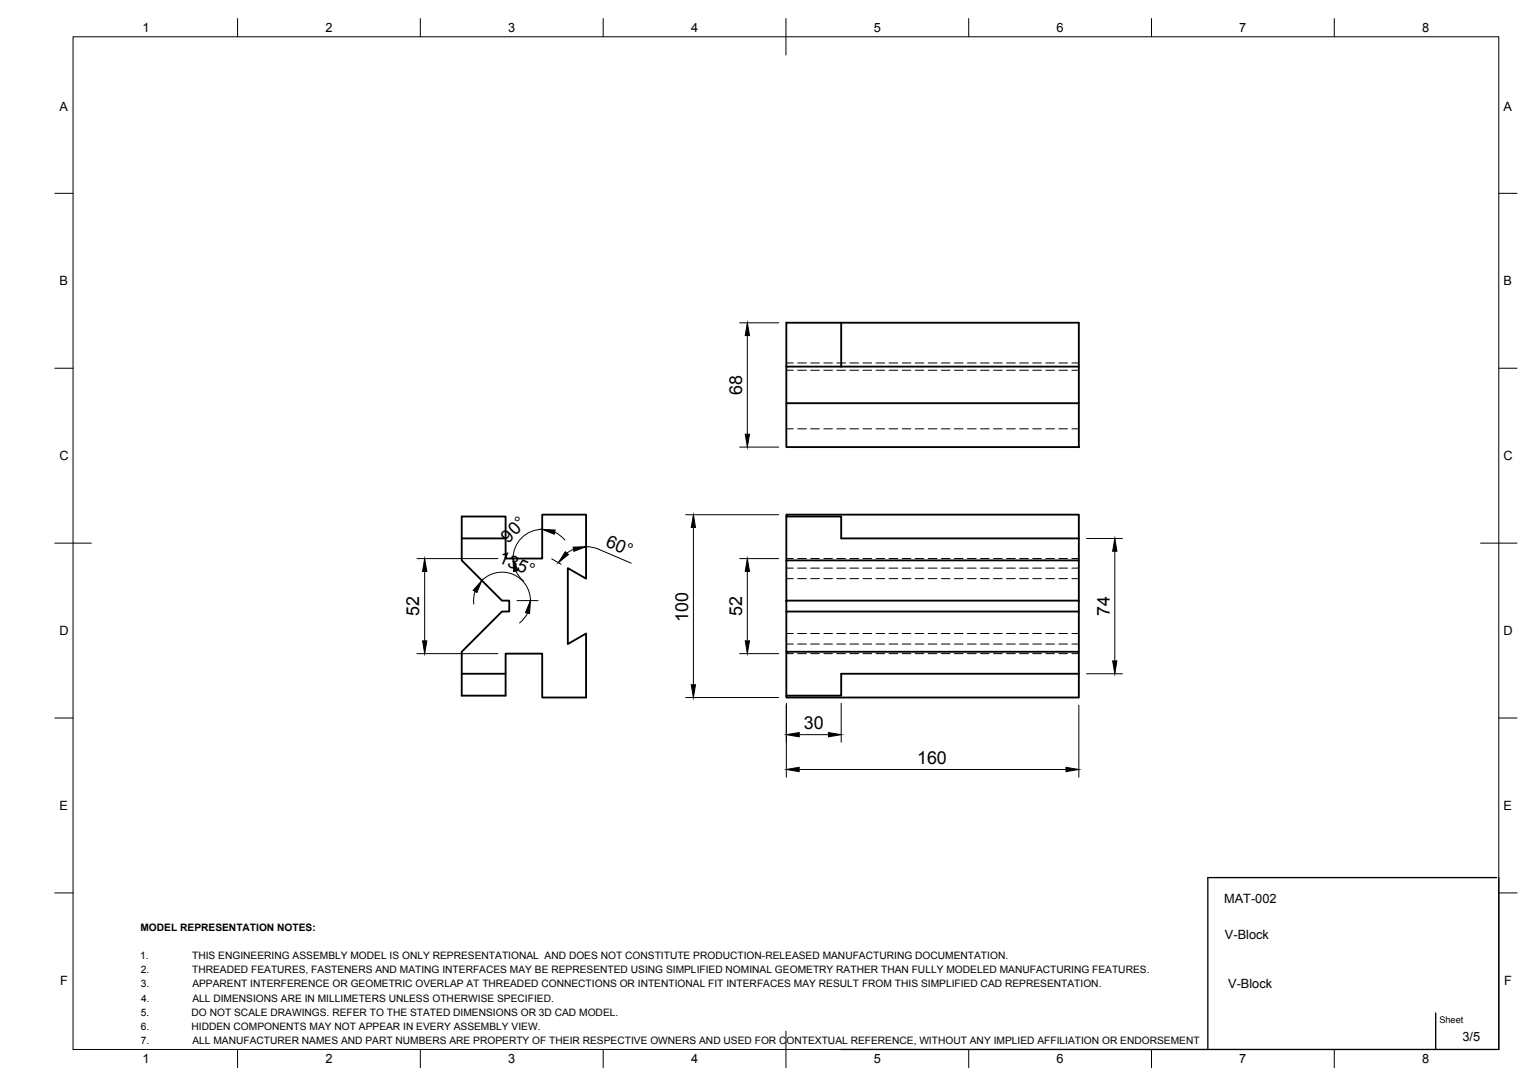
ISO-10303-21;
HEADER;
/* Generated by software containing ST-Developer
 * from STEP Tools, Inc. (www.steptools.com) 
 */

FILE_DESCRIPTION(
/* description */ ('STEP AP214'),
/* implementation_level */ '2;1');

FILE_NAME(
/* name */ 'V-Block.step',
/* time_stamp */ '2026-11-14T04:35:10-08:00',
/* author */ (''),
/* organization */ (''),
/* preprocessor_version */ 'ST-DEVELOPER v20.2',
/* originating_system */ 'Autodesk Translation Framework v15.17.0.0',
/* authorisation */ '');

FILE_SCHEMA (('AUTOMOTIVE_DESIGN { 1 0 10303 214 3 1 1 }'));
ENDSEC;

DATA;
#10=MECHANICAL_DESIGN_GEOMETRIC_PRESENTATION_REPRESENTATION('',(#107),#2477);
#99=SHAPE_REPRESENTATION_RELATIONSHIP('SRR','None',#2497,#103);
#103=ADVANCED_BREP_SHAPE_REPRESENTATION('',(#111),#2473);
#107=STYLED_ITEM('',(#2526),#111);
#111=MANIFOLD_SOLID_BREP('Body1',#1427);
#115=FACE_OUTER_BOUND('',#194,.T.);
#116=FACE_OUTER_BOUND('',#195,.T.);
#117=FACE_OUTER_BOUND('',#196,.T.);
#118=FACE_OUTER_BOUND('',#197,.T.);
#119=FACE_OUTER_BOUND('',#198,.T.);
#120=FACE_OUTER_BOUND('',#199,.T.);
#121=FACE_OUTER_BOUND('',#200,.T.);
#122=FACE_OUTER_BOUND('',#201,.T.);
#123=FACE_OUTER_BOUND('',#202,.T.);
#124=FACE_OUTER_BOUND('',#203,.T.);
#125=FACE_OUTER_BOUND('',#204,.T.);
#126=FACE_OUTER_BOUND('',#205,.T.);
#127=FACE_OUTER_BOUND('',#206,.T.);
#128=FACE_OUTER_BOUND('',#207,.T.);
#129=FACE_OUTER_BOUND('',#208,.T.);
#130=FACE_OUTER_BOUND('',#209,.T.);
#131=FACE_OUTER_BOUND('',#210,.T.);
#132=FACE_OUTER_BOUND('',#211,.T.);
#133=FACE_OUTER_BOUND('',#212,.T.);
#134=FACE_OUTER_BOUND('',#213,.T.);
#135=FACE_OUTER_BOUND('',#214,.T.);
#136=FACE_OUTER_BOUND('',#215,.T.);
#137=FACE_OUTER_BOUND('',#216,.T.);
#138=FACE_OUTER_BOUND('',#217,.T.);
#139=FACE_OUTER_BOUND('',#218,.T.);
#140=FACE_OUTER_BOUND('',#219,.T.);
#141=FACE_OUTER_BOUND('',#220,.T.);
#142=FACE_OUTER_BOUND('',#221,.T.);
#194=EDGE_LOOP('',(#894,#895,#896,#897));
#195=EDGE_LOOP('',(#898,#899,#900,#901));
#196=EDGE_LOOP('',(#902,#903,#904,#905));
#197=EDGE_LOOP('',(#906,#907,#908,#909));
#198=EDGE_LOOP('',(#910,#911,#912,#913));
#199=EDGE_LOOP('',(#914,#915,#916,#917,#918,#919));
#200=EDGE_LOOP('',(#920,#921,#922,#923,#924,#925));
#201=EDGE_LOOP('',(#926,#927,#928,#929));
#202=EDGE_LOOP('',(#930,#931,#932,#933));
#203=EDGE_LOOP('',(#934,#935,#936,#937));
#204=EDGE_LOOP('',(#938,#939,#940,#941));
#205=EDGE_LOOP('',(#942,#943,#944,#945));
#206=EDGE_LOOP('',(#946,#947,#948,#949,#950,#951));
#207=EDGE_LOOP('',(#952,#953,#954,#955,#956,#957));
#208=EDGE_LOOP('',(#958,#959,#960,#961));
#209=EDGE_LOOP('',(#962,#963,#964,#965));
#210=EDGE_LOOP('',(#966,#967,#968,#969));
#211=EDGE_LOOP('',(#970,#971,#972,#973));
#212=EDGE_LOOP('',(#974,#975,#976,#977));
#213=EDGE_LOOP('',(#978,#979,#980,#981));
#214=EDGE_LOOP('',(#982,#983,#984,#985));
#215=EDGE_LOOP('',(#986,#987,#988,#989));
#216=EDGE_LOOP('',(#990,#991,#992,#993,#994,#995,#996,#997,#998,#999,#1000,
#1001,#1002,#1003,#1004,#1005,#1006,#1007,#1008,#1009,#1010,#1011));
#217=EDGE_LOOP('',(#1012,#1013,#1014,#1015,#1016,#1017,#1018,#1019,#1020,
#1021,#1022,#1023,#1024,#1025,#1026,#1027,#1028,#1029,#1030,#1031,#1032,
#1033));
#218=EDGE_LOOP('',(#1034,#1035,#1036,#1037));
#219=EDGE_LOOP('',(#1038,#1039,#1040,#1041));
#220=EDGE_LOOP('',(#1042,#1043,#1044,#1045));
#221=EDGE_LOOP('',(#1046,#1047,#1048,#1049));
#276=LINE('',#2000,#423);
#277=LINE('',#2002,#424);
#278=LINE('',#2004,#425);
#279=LINE('',#2005,#426);
#280=LINE('',#2009,#427);
#281=LINE('',#2011,#428);
#282=LINE('',#2013,#429);
#283=LINE('',#2014,#430);
#284=LINE('',#2018,#431);
#285=LINE('',#2020,#432);
#286=LINE('',#2022,#433);
#287=LINE('',#2023,#434);
#288=LINE('',#2026,#435);
#289=LINE('',#2028,#436);
#290=LINE('',#2029,#437);
#291=LINE('',#2032,#438);
#292=LINE('',#2034,#439);
#293=LINE('',#2035,#440);
#294=LINE('',#2037,#441);
#295=LINE('',#2039,#442);
#296=LINE('',#2041,#443);
#297=LINE('',#2042,#444);
#298=LINE('',#2045,#445);
#299=LINE('',#2047,#446);
#300=LINE('',#2049,#447);
#301=LINE('',#2051,#448);
#302=LINE('',#2052,#449);
#303=LINE('',#2055,#450);
#304=LINE('',#2057,#451);
#305=LINE('',#2058,#452);
#306=LINE('',#2061,#453);
#307=LINE('',#2063,#454);
#308=LINE('',#2064,#455);
#309=LINE('',#2067,#456);
#310=LINE('',#2069,#457);
#311=LINE('',#2070,#458);
#312=LINE('',#2073,#459);
#313=LINE('',#2075,#460);
#314=LINE('',#2076,#461);
#315=LINE('',#2079,#462);
#316=LINE('',#2081,#463);
#317=LINE('',#2082,#464);
#318=LINE('',#2084,#465);
#319=LINE('',#2086,#466);
#320=LINE('',#2088,#467);
#321=LINE('',#2089,#468);
#322=LINE('',#2092,#469);
#323=LINE('',#2094,#470);
#324=LINE('',#2096,#471);
#325=LINE('',#2098,#472);
#326=LINE('',#2099,#473);
#327=LINE('',#2102,#474);
#328=LINE('',#2104,#475);
#329=LINE('',#2105,#476);
#330=LINE('',#2108,#477);
#331=LINE('',#2110,#478);
#332=LINE('',#2111,#479);
#333=LINE('',#2114,#480);
#334=LINE('',#2116,#481);
#335=LINE('',#2117,#482);
#336=LINE('',#2120,#483);
#337=LINE('',#2122,#484);
#338=LINE('',#2123,#485);
#339=LINE('',#2126,#486);
#340=LINE('',#2128,#487);
#341=LINE('',#2129,#488);
#342=LINE('',#2132,#489);
#343=LINE('',#2134,#490);
#344=LINE('',#2135,#491);
#345=LINE('',#2138,#492);
#346=LINE('',#2140,#493);
#347=LINE('',#2141,#494);
#348=LINE('',#2143,#495);
#349=LINE('',#2144,#496);
#350=LINE('',#2146,#497);
#351=LINE('',#2147,#498);
#352=LINE('',#2150,#499);
#353=LINE('',#2153,#500);
#423=VECTOR('',#1606,1000.);
#424=VECTOR('',#1607,1000.);
#425=VECTOR('',#1608,1000.);
#426=VECTOR('',#1609,1000.);
#427=VECTOR('',#1612,1000.);
#428=VECTOR('',#1613,1000.);
#429=VECTOR('',#1614,1000.);
#430=VECTOR('',#1615,1000.);
#431=VECTOR('',#1618,1000.);
#432=VECTOR('',#1619,1000.);
#433=VECTOR('',#1620,1000.);
#434=VECTOR('',#1621,1000.);
#435=VECTOR('',#1624,1000.);
#436=VECTOR('',#1625,1000.);
#437=VECTOR('',#1626,1000.);
#438=VECTOR('',#1629,1000.);
#439=VECTOR('',#1630,1000.);
#440=VECTOR('',#1631,1000.);
#441=VECTOR('',#1634,1000.);
#442=VECTOR('',#1635,1000.);
#443=VECTOR('',#1636,1000.);
#444=VECTOR('',#1637,1000.);
#445=VECTOR('',#1640,1000.);
#446=VECTOR('',#1641,1000.);
#447=VECTOR('',#1642,1000.);
#448=VECTOR('',#1643,1000.);
#449=VECTOR('',#1644,1000.);
#450=VECTOR('',#1647,1000.);
#451=VECTOR('',#1648,1000.);
#452=VECTOR('',#1649,1000.);
#453=VECTOR('',#1652,1000.);
#454=VECTOR('',#1653,1000.);
#455=VECTOR('',#1654,1000.);
#456=VECTOR('',#1657,1000.);
#457=VECTOR('',#1658,1000.);
#458=VECTOR('',#1659,1000.);
#459=VECTOR('',#1662,1000.);
#460=VECTOR('',#1663,1000.);
#461=VECTOR('',#1664,1000.);
#462=VECTOR('',#1667,1000.);
#463=VECTOR('',#1668,1000.);
#464=VECTOR('',#1669,1000.);
#465=VECTOR('',#1672,1000.);
#466=VECTOR('',#1673,1000.);
#467=VECTOR('',#1674,1000.);
#468=VECTOR('',#1675,1000.);
#469=VECTOR('',#1678,1000.);
#470=VECTOR('',#1679,1000.);
#471=VECTOR('',#1680,1000.);
#472=VECTOR('',#1681,1000.);
#473=VECTOR('',#1682,1000.);
#474=VECTOR('',#1685,1000.);
#475=VECTOR('',#1686,1000.);
#476=VECTOR('',#1687,1000.);
#477=VECTOR('',#1690,1000.);
#478=VECTOR('',#1691,1000.);
#479=VECTOR('',#1692,1000.);
#480=VECTOR('',#1695,1000.);
#481=VECTOR('',#1696,1000.);
#482=VECTOR('',#1697,1000.);
#483=VECTOR('',#1700,1000.);
#484=VECTOR('',#1701,1000.);
#485=VECTOR('',#1702,1000.);
#486=VECTOR('',#1705,1000.);
#487=VECTOR('',#1706,1000.);
#488=VECTOR('',#1707,1000.);
#489=VECTOR('',#1710,1000.);
#490=VECTOR('',#1711,1000.);
#491=VECTOR('',#1712,1000.);
#492=VECTOR('',#1715,1000.);
#493=VECTOR('',#1716,1000.);
#494=VECTOR('',#1717,1000.);
#495=VECTOR('',#1720,1000.);
#496=VECTOR('',#1721,1000.);
#497=VECTOR('',#1724,1000.);
#498=VECTOR('',#1725,1000.);
#499=VECTOR('',#1730,1000.);
#500=VECTOR('',#1735,1000.);
#570=VERTEX_POINT('',#1998);
#571=VERTEX_POINT('',#1999);
#572=VERTEX_POINT('',#2001);
#573=VERTEX_POINT('',#2003);
#574=VERTEX_POINT('',#2007);
#575=VERTEX_POINT('',#2008);
#576=VERTEX_POINT('',#2010);
#577=VERTEX_POINT('',#2012);
#578=VERTEX_POINT('',#2016);
#579=VERTEX_POINT('',#2017);
#580=VERTEX_POINT('',#2019);
#581=VERTEX_POINT('',#2021);
#582=VERTEX_POINT('',#2025);
#583=VERTEX_POINT('',#2027);
#584=VERTEX_POINT('',#2031);
#585=VERTEX_POINT('',#2033);
#586=VERTEX_POINT('',#2038);
#587=VERTEX_POINT('',#2040);
#588=VERTEX_POINT('',#2044);
#589=VERTEX_POINT('',#2046);
#590=VERTEX_POINT('',#2048);
#591=VERTEX_POINT('',#2050);
#592=VERTEX_POINT('',#2054);
#593=VERTEX_POINT('',#2056);
#594=VERTEX_POINT('',#2060);
#595=VERTEX_POINT('',#2062);
#596=VERTEX_POINT('',#2066);
#597=VERTEX_POINT('',#2068);
#598=VERTEX_POINT('',#2072);
#599=VERTEX_POINT('',#2074);
#600=VERTEX_POINT('',#2078);
#601=VERTEX_POINT('',#2080);
#602=VERTEX_POINT('',#2085);
#603=VERTEX_POINT('',#2087);
#604=VERTEX_POINT('',#2091);
#605=VERTEX_POINT('',#2093);
#606=VERTEX_POINT('',#2095);
#607=VERTEX_POINT('',#2097);
#608=VERTEX_POINT('',#2101);
#609=VERTEX_POINT('',#2103);
#610=VERTEX_POINT('',#2107);
#611=VERTEX_POINT('',#2109);
#612=VERTEX_POINT('',#2113);
#613=VERTEX_POINT('',#2115);
#614=VERTEX_POINT('',#2119);
#615=VERTEX_POINT('',#2121);
#616=VERTEX_POINT('',#2125);
#617=VERTEX_POINT('',#2127);
#618=VERTEX_POINT('',#2131);
#619=VERTEX_POINT('',#2133);
#620=VERTEX_POINT('',#2137);
#621=VERTEX_POINT('',#2139);
#697=EDGE_CURVE('',#570,#571,#276,.T.);
#698=EDGE_CURVE('',#572,#570,#277,.T.);
#699=EDGE_CURVE('',#572,#573,#278,.T.);
#700=EDGE_CURVE('',#571,#573,#279,.T.);
#701=EDGE_CURVE('',#574,#575,#280,.T.);
#702=EDGE_CURVE('',#576,#574,#281,.T.);
#703=EDGE_CURVE('',#576,#577,#282,.T.);
#704=EDGE_CURVE('',#575,#577,#283,.T.);
#705=EDGE_CURVE('',#578,#579,#284,.T.);
#706=EDGE_CURVE('',#580,#578,#285,.T.);
#707=EDGE_CURVE('',#580,#581,#286,.T.);
#708=EDGE_CURVE('',#581,#579,#287,.T.);
#709=EDGE_CURVE('',#582,#578,#288,.T.);
#710=EDGE_CURVE('',#583,#582,#289,.T.);
#711=EDGE_CURVE('',#583,#580,#290,.T.);
#712=EDGE_CURVE('',#584,#582,#291,.T.);
#713=EDGE_CURVE('',#585,#584,#292,.T.);
#714=EDGE_CURVE('',#585,#583,#293,.T.);
#715=EDGE_CURVE('',#573,#584,#294,.T.);
#716=EDGE_CURVE('',#586,#572,#295,.T.);
#717=EDGE_CURVE('',#587,#586,#296,.T.);
#718=EDGE_CURVE('',#587,#585,#297,.T.);
#719=EDGE_CURVE('',#588,#571,#298,.T.);
#720=EDGE_CURVE('',#589,#588,#299,.T.);
#721=EDGE_CURVE('',#589,#590,#300,.T.);
#722=EDGE_CURVE('',#591,#590,#301,.T.);
#723=EDGE_CURVE('',#591,#570,#302,.T.);
#724=EDGE_CURVE('',#592,#588,#303,.T.);
#725=EDGE_CURVE('',#593,#592,#304,.T.);
#726=EDGE_CURVE('',#593,#589,#305,.T.);
#727=EDGE_CURVE('',#594,#592,#306,.T.);
#728=EDGE_CURVE('',#595,#594,#307,.T.);
#729=EDGE_CURVE('',#595,#593,#308,.T.);
#730=EDGE_CURVE('',#596,#594,#309,.T.);
#731=EDGE_CURVE('',#597,#596,#310,.T.);
#732=EDGE_CURVE('',#597,#595,#311,.T.);
#733=EDGE_CURVE('',#598,#596,#312,.T.);
#734=EDGE_CURVE('',#599,#598,#313,.T.);
#735=EDGE_CURVE('',#599,#597,#314,.T.);
#736=EDGE_CURVE('',#600,#598,#315,.T.);
#737=EDGE_CURVE('',#601,#600,#316,.T.);
#738=EDGE_CURVE('',#601,#599,#317,.T.);
#739=EDGE_CURVE('',#577,#600,#318,.T.);
#740=EDGE_CURVE('',#602,#576,#319,.T.);
#741=EDGE_CURVE('',#603,#602,#320,.T.);
#742=EDGE_CURVE('',#603,#601,#321,.T.);
#743=EDGE_CURVE('',#604,#575,#322,.T.);
#744=EDGE_CURVE('',#605,#604,#323,.T.);
#745=EDGE_CURVE('',#605,#606,#324,.T.);
#746=EDGE_CURVE('',#607,#606,#325,.T.);
#747=EDGE_CURVE('',#607,#574,#326,.T.);
#748=EDGE_CURVE('',#608,#604,#327,.T.);
#749=EDGE_CURVE('',#609,#608,#328,.T.);
#750=EDGE_CURVE('',#609,#605,#329,.T.);
#751=EDGE_CURVE('',#610,#608,#330,.T.);
#752=EDGE_CURVE('',#611,#610,#331,.T.);
#753=EDGE_CURVE('',#611,#609,#332,.T.);
#754=EDGE_CURVE('',#612,#610,#333,.T.);
#755=EDGE_CURVE('',#613,#612,#334,.T.);
#756=EDGE_CURVE('',#613,#611,#335,.T.);
#757=EDGE_CURVE('',#614,#612,#336,.T.);
#758=EDGE_CURVE('',#615,#614,#337,.T.);
#759=EDGE_CURVE('',#615,#613,#338,.T.);
#760=EDGE_CURVE('',#616,#614,#339,.T.);
#761=EDGE_CURVE('',#617,#616,#340,.T.);
#762=EDGE_CURVE('',#617,#615,#341,.T.);
#763=EDGE_CURVE('',#618,#616,#342,.T.);
#764=EDGE_CURVE('',#619,#618,#343,.T.);
#765=EDGE_CURVE('',#619,#617,#344,.T.);
#766=EDGE_CURVE('',#620,#618,#345,.T.);
#767=EDGE_CURVE('',#621,#620,#346,.T.);
#768=EDGE_CURVE('',#621,#619,#347,.T.);
#769=EDGE_CURVE('',#579,#620,#348,.T.);
#770=EDGE_CURVE('',#581,#621,#349,.T.);
#771=EDGE_CURVE('',#590,#587,#350,.T.);
#772=EDGE_CURVE('',#606,#603,#351,.T.);
#773=EDGE_CURVE('',#602,#607,#352,.T.);
#774=EDGE_CURVE('',#586,#591,#353,.T.);
#894=ORIENTED_EDGE('',*,*,#697,.F.);
#895=ORIENTED_EDGE('',*,*,#698,.F.);
#896=ORIENTED_EDGE('',*,*,#699,.T.);
#897=ORIENTED_EDGE('',*,*,#700,.F.);
#898=ORIENTED_EDGE('',*,*,#701,.F.);
#899=ORIENTED_EDGE('',*,*,#702,.F.);
#900=ORIENTED_EDGE('',*,*,#703,.T.);
#901=ORIENTED_EDGE('',*,*,#704,.F.);
#902=ORIENTED_EDGE('',*,*,#705,.F.);
#903=ORIENTED_EDGE('',*,*,#706,.F.);
#904=ORIENTED_EDGE('',*,*,#707,.T.);
#905=ORIENTED_EDGE('',*,*,#708,.T.);
#906=ORIENTED_EDGE('',*,*,#709,.F.);
#907=ORIENTED_EDGE('',*,*,#710,.F.);
#908=ORIENTED_EDGE('',*,*,#711,.T.);
#909=ORIENTED_EDGE('',*,*,#706,.T.);
#910=ORIENTED_EDGE('',*,*,#712,.F.);
#911=ORIENTED_EDGE('',*,*,#713,.F.);
#912=ORIENTED_EDGE('',*,*,#714,.T.);
#913=ORIENTED_EDGE('',*,*,#710,.T.);
#914=ORIENTED_EDGE('',*,*,#715,.F.);
#915=ORIENTED_EDGE('',*,*,#699,.F.);
#916=ORIENTED_EDGE('',*,*,#716,.F.);
#917=ORIENTED_EDGE('',*,*,#717,.F.);
#918=ORIENTED_EDGE('',*,*,#718,.T.);
#919=ORIENTED_EDGE('',*,*,#713,.T.);
#920=ORIENTED_EDGE('',*,*,#719,.F.);
#921=ORIENTED_EDGE('',*,*,#720,.F.);
#922=ORIENTED_EDGE('',*,*,#721,.T.);
#923=ORIENTED_EDGE('',*,*,#722,.F.);
#924=ORIENTED_EDGE('',*,*,#723,.T.);
#925=ORIENTED_EDGE('',*,*,#697,.T.);
#926=ORIENTED_EDGE('',*,*,#724,.F.);
#927=ORIENTED_EDGE('',*,*,#725,.F.);
#928=ORIENTED_EDGE('',*,*,#726,.T.);
#929=ORIENTED_EDGE('',*,*,#720,.T.);
#930=ORIENTED_EDGE('',*,*,#727,.F.);
#931=ORIENTED_EDGE('',*,*,#728,.F.);
#932=ORIENTED_EDGE('',*,*,#729,.T.);
#933=ORIENTED_EDGE('',*,*,#725,.T.);
#934=ORIENTED_EDGE('',*,*,#730,.F.);
#935=ORIENTED_EDGE('',*,*,#731,.F.);
#936=ORIENTED_EDGE('',*,*,#732,.T.);
#937=ORIENTED_EDGE('',*,*,#728,.T.);
#938=ORIENTED_EDGE('',*,*,#733,.F.);
#939=ORIENTED_EDGE('',*,*,#734,.F.);
#940=ORIENTED_EDGE('',*,*,#735,.T.);
#941=ORIENTED_EDGE('',*,*,#731,.T.);
#942=ORIENTED_EDGE('',*,*,#736,.F.);
#943=ORIENTED_EDGE('',*,*,#737,.F.);
#944=ORIENTED_EDGE('',*,*,#738,.T.);
#945=ORIENTED_EDGE('',*,*,#734,.T.);
#946=ORIENTED_EDGE('',*,*,#739,.F.);
#947=ORIENTED_EDGE('',*,*,#703,.F.);
#948=ORIENTED_EDGE('',*,*,#740,.F.);
#949=ORIENTED_EDGE('',*,*,#741,.F.);
#950=ORIENTED_EDGE('',*,*,#742,.T.);
#951=ORIENTED_EDGE('',*,*,#737,.T.);
#952=ORIENTED_EDGE('',*,*,#743,.F.);
#953=ORIENTED_EDGE('',*,*,#744,.F.);
#954=ORIENTED_EDGE('',*,*,#745,.T.);
#955=ORIENTED_EDGE('',*,*,#746,.F.);
#956=ORIENTED_EDGE('',*,*,#747,.T.);
#957=ORIENTED_EDGE('',*,*,#701,.T.);
#958=ORIENTED_EDGE('',*,*,#748,.F.);
#959=ORIENTED_EDGE('',*,*,#749,.F.);
#960=ORIENTED_EDGE('',*,*,#750,.T.);
#961=ORIENTED_EDGE('',*,*,#744,.T.);
#962=ORIENTED_EDGE('',*,*,#751,.F.);
#963=ORIENTED_EDGE('',*,*,#752,.F.);
#964=ORIENTED_EDGE('',*,*,#753,.T.);
#965=ORIENTED_EDGE('',*,*,#749,.T.);
#966=ORIENTED_EDGE('',*,*,#754,.F.);
#967=ORIENTED_EDGE('',*,*,#755,.F.);
#968=ORIENTED_EDGE('',*,*,#756,.T.);
#969=ORIENTED_EDGE('',*,*,#752,.T.);
#970=ORIENTED_EDGE('',*,*,#757,.F.);
#971=ORIENTED_EDGE('',*,*,#758,.F.);
#972=ORIENTED_EDGE('',*,*,#759,.T.);
#973=ORIENTED_EDGE('',*,*,#755,.T.);
#974=ORIENTED_EDGE('',*,*,#760,.F.);
#975=ORIENTED_EDGE('',*,*,#761,.F.);
#976=ORIENTED_EDGE('',*,*,#762,.T.);
#977=ORIENTED_EDGE('',*,*,#758,.T.);
#978=ORIENTED_EDGE('',*,*,#763,.F.);
#979=ORIENTED_EDGE('',*,*,#764,.F.);
#980=ORIENTED_EDGE('',*,*,#765,.T.);
#981=ORIENTED_EDGE('',*,*,#761,.T.);
#982=ORIENTED_EDGE('',*,*,#766,.F.);
#983=ORIENTED_EDGE('',*,*,#767,.F.);
#984=ORIENTED_EDGE('',*,*,#768,.T.);
#985=ORIENTED_EDGE('',*,*,#764,.T.);
#986=ORIENTED_EDGE('',*,*,#769,.F.);
#987=ORIENTED_EDGE('',*,*,#708,.F.);
#988=ORIENTED_EDGE('',*,*,#770,.T.);
#989=ORIENTED_EDGE('',*,*,#767,.T.);
#990=ORIENTED_EDGE('',*,*,#707,.F.);
#991=ORIENTED_EDGE('',*,*,#711,.F.);
#992=ORIENTED_EDGE('',*,*,#714,.F.);
#993=ORIENTED_EDGE('',*,*,#718,.F.);
#994=ORIENTED_EDGE('',*,*,#771,.F.);
#995=ORIENTED_EDGE('',*,*,#721,.F.);
#996=ORIENTED_EDGE('',*,*,#726,.F.);
#997=ORIENTED_EDGE('',*,*,#729,.F.);
#998=ORIENTED_EDGE('',*,*,#732,.F.);
#999=ORIENTED_EDGE('',*,*,#735,.F.);
#1000=ORIENTED_EDGE('',*,*,#738,.F.);
#1001=ORIENTED_EDGE('',*,*,#742,.F.);
#1002=ORIENTED_EDGE('',*,*,#772,.F.);
#1003=ORIENTED_EDGE('',*,*,#745,.F.);
#1004=ORIENTED_EDGE('',*,*,#750,.F.);
#1005=ORIENTED_EDGE('',*,*,#753,.F.);
#1006=ORIENTED_EDGE('',*,*,#756,.F.);
#1007=ORIENTED_EDGE('',*,*,#759,.F.);
#1008=ORIENTED_EDGE('',*,*,#762,.F.);
#1009=ORIENTED_EDGE('',*,*,#765,.F.);
#1010=ORIENTED_EDGE('',*,*,#768,.F.);
#1011=ORIENTED_EDGE('',*,*,#770,.F.);
#1012=ORIENTED_EDGE('',*,*,#705,.T.);
#1013=ORIENTED_EDGE('',*,*,#769,.T.);
#1014=ORIENTED_EDGE('',*,*,#766,.T.);
#1015=ORIENTED_EDGE('',*,*,#763,.T.);
#1016=ORIENTED_EDGE('',*,*,#760,.T.);
#1017=ORIENTED_EDGE('',*,*,#757,.T.);
#1018=ORIENTED_EDGE('',*,*,#754,.T.);
#1019=ORIENTED_EDGE('',*,*,#751,.T.);
#1020=ORIENTED_EDGE('',*,*,#748,.T.);
#1021=ORIENTED_EDGE('',*,*,#743,.T.);
#1022=ORIENTED_EDGE('',*,*,#704,.T.);
#1023=ORIENTED_EDGE('',*,*,#739,.T.);
#1024=ORIENTED_EDGE('',*,*,#736,.T.);
#1025=ORIENTED_EDGE('',*,*,#733,.T.);
#1026=ORIENTED_EDGE('',*,*,#730,.T.);
#1027=ORIENTED_EDGE('',*,*,#727,.T.);
#1028=ORIENTED_EDGE('',*,*,#724,.T.);
#1029=ORIENTED_EDGE('',*,*,#719,.T.);
#1030=ORIENTED_EDGE('',*,*,#700,.T.);
#1031=ORIENTED_EDGE('',*,*,#715,.T.);
#1032=ORIENTED_EDGE('',*,*,#712,.T.);
#1033=ORIENTED_EDGE('',*,*,#709,.T.);
#1034=ORIENTED_EDGE('',*,*,#702,.T.);
#1035=ORIENTED_EDGE('',*,*,#747,.F.);
#1036=ORIENTED_EDGE('',*,*,#773,.F.);
#1037=ORIENTED_EDGE('',*,*,#740,.T.);
#1038=ORIENTED_EDGE('',*,*,#772,.T.);
#1039=ORIENTED_EDGE('',*,*,#741,.T.);
#1040=ORIENTED_EDGE('',*,*,#773,.T.);
#1041=ORIENTED_EDGE('',*,*,#746,.T.);
#1042=ORIENTED_EDGE('',*,*,#698,.T.);
#1043=ORIENTED_EDGE('',*,*,#723,.F.);
#1044=ORIENTED_EDGE('',*,*,#774,.F.);
#1045=ORIENTED_EDGE('',*,*,#716,.T.);
#1046=ORIENTED_EDGE('',*,*,#771,.T.);
#1047=ORIENTED_EDGE('',*,*,#717,.T.);
#1048=ORIENTED_EDGE('',*,*,#774,.T.);
#1049=ORIENTED_EDGE('',*,*,#722,.T.);
#1288=PLANE('',#1478);
#1289=PLANE('',#1479);
#1290=PLANE('',#1480);
#1291=PLANE('',#1481);
#1292=PLANE('',#1482);
#1293=PLANE('',#1483);
#1294=PLANE('',#1484);
#1295=PLANE('',#1485);
#1296=PLANE('',#1486);
#1297=PLANE('',#1487);
#1298=PLANE('',#1488);
#1299=PLANE('',#1489);
#1300=PLANE('',#1490);
#1301=PLANE('',#1491);
#1302=PLANE('',#1492);
#1303=PLANE('',#1493);
#1304=PLANE('',#1494);
#1305=PLANE('',#1495);
#1306=PLANE('',#1496);
#1307=PLANE('',#1497);
#1308=PLANE('',#1498);
#1309=PLANE('',#1499);
#1310=PLANE('',#1500);
#1311=PLANE('',#1501);
#1312=PLANE('',#1502);
#1313=PLANE('',#1503);
#1314=PLANE('',#1504);
#1315=PLANE('',#1505);
#1348=ADVANCED_FACE('',(#115),#1288,.T.);
#1349=ADVANCED_FACE('',(#116),#1289,.T.);
#1350=ADVANCED_FACE('',(#117),#1290,.T.);
#1351=ADVANCED_FACE('',(#118),#1291,.T.);
#1352=ADVANCED_FACE('',(#119),#1292,.T.);
#1353=ADVANCED_FACE('',(#120),#1293,.T.);
#1354=ADVANCED_FACE('',(#121),#1294,.T.);
#1355=ADVANCED_FACE('',(#122),#1295,.T.);
#1356=ADVANCED_FACE('',(#123),#1296,.T.);
#1357=ADVANCED_FACE('',(#124),#1297,.T.);
#1358=ADVANCED_FACE('',(#125),#1298,.T.);
#1359=ADVANCED_FACE('',(#126),#1299,.T.);
#1360=ADVANCED_FACE('',(#127),#1300,.T.);
#1361=ADVANCED_FACE('',(#128),#1301,.T.);
#1362=ADVANCED_FACE('',(#129),#1302,.T.);
#1363=ADVANCED_FACE('',(#130),#1303,.T.);
#1364=ADVANCED_FACE('',(#131),#1304,.T.);
#1365=ADVANCED_FACE('',(#132),#1305,.T.);
#1366=ADVANCED_FACE('',(#133),#1306,.T.);
#1367=ADVANCED_FACE('',(#134),#1307,.T.);
#1368=ADVANCED_FACE('',(#135),#1308,.T.);
#1369=ADVANCED_FACE('',(#136),#1309,.T.);
#1370=ADVANCED_FACE('',(#137),#1310,.T.);
#1371=ADVANCED_FACE('',(#138),#1311,.F.);
#1372=ADVANCED_FACE('',(#139),#1312,.F.);
#1373=ADVANCED_FACE('',(#140),#1313,.T.);
#1374=ADVANCED_FACE('',(#141),#1314,.F.);
#1375=ADVANCED_FACE('',(#142),#1315,.F.);
#1427=CLOSED_SHELL('',(#1348,#1349,#1350,#1351,#1352,#1353,#1354,#1355,
#1356,#1357,#1358,#1359,#1360,#1361,#1362,#1363,#1364,#1365,#1366,#1367,
#1368,#1369,#1370,#1371,#1372,#1373,#1374,#1375));
#1477=AXIS2_PLACEMENT_3D('',#1996,#1602,#1603);
#1478=AXIS2_PLACEMENT_3D('',#1997,#1604,#1605);
#1479=AXIS2_PLACEMENT_3D('',#2006,#1610,#1611);
#1480=AXIS2_PLACEMENT_3D('',#2015,#1616,#1617);
#1481=AXIS2_PLACEMENT_3D('',#2024,#1622,#1623);
#1482=AXIS2_PLACEMENT_3D('',#2030,#1627,#1628);
#1483=AXIS2_PLACEMENT_3D('',#2036,#1632,#1633);
#1484=AXIS2_PLACEMENT_3D('',#2043,#1638,#1639);
#1485=AXIS2_PLACEMENT_3D('',#2053,#1645,#1646);
#1486=AXIS2_PLACEMENT_3D('',#2059,#1650,#1651);
#1487=AXIS2_PLACEMENT_3D('',#2065,#1655,#1656);
#1488=AXIS2_PLACEMENT_3D('',#2071,#1660,#1661);
#1489=AXIS2_PLACEMENT_3D('',#2077,#1665,#1666);
#1490=AXIS2_PLACEMENT_3D('',#2083,#1670,#1671);
#1491=AXIS2_PLACEMENT_3D('',#2090,#1676,#1677);
#1492=AXIS2_PLACEMENT_3D('',#2100,#1683,#1684);
#1493=AXIS2_PLACEMENT_3D('',#2106,#1688,#1689);
#1494=AXIS2_PLACEMENT_3D('',#2112,#1693,#1694);
#1495=AXIS2_PLACEMENT_3D('',#2118,#1698,#1699);
#1496=AXIS2_PLACEMENT_3D('',#2124,#1703,#1704);
#1497=AXIS2_PLACEMENT_3D('',#2130,#1708,#1709);
#1498=AXIS2_PLACEMENT_3D('',#2136,#1713,#1714);
#1499=AXIS2_PLACEMENT_3D('',#2142,#1718,#1719);
#1500=AXIS2_PLACEMENT_3D('',#2145,#1722,#1723);
#1501=AXIS2_PLACEMENT_3D('',#2148,#1726,#1727);
#1502=AXIS2_PLACEMENT_3D('',#2149,#1728,#1729);
#1503=AXIS2_PLACEMENT_3D('',#2151,#1731,#1732);
#1504=AXIS2_PLACEMENT_3D('',#2152,#1733,#1734);
#1505=AXIS2_PLACEMENT_3D('',#2154,#1736,#1737);
#1602=DIRECTION('axis',(0.,0.,1.));
#1603=DIRECTION('refdir',(1.,0.,0.));
#1604=DIRECTION('center_axis',(-1.,0.,0.));
#1605=DIRECTION('ref_axis',(0.,0.,1.));
#1606=DIRECTION('',(0.,0.,1.));
#1607=DIRECTION('',(0.,1.,0.));
#1608=DIRECTION('',(0.,0.,1.));
#1609=DIRECTION('',(0.,-1.,0.));
#1610=DIRECTION('center_axis',(1.,0.,0.));
#1611=DIRECTION('ref_axis',(0.,0.,-1.));
#1612=DIRECTION('',(0.,0.,1.));
#1613=DIRECTION('',(0.,-1.,0.));
#1614=DIRECTION('',(0.,0.,1.));
#1615=DIRECTION('',(0.,1.,0.));
#1616=DIRECTION('center_axis',(-1.,0.,0.));
#1617=DIRECTION('ref_axis',(0.,0.,1.));
#1618=DIRECTION('',(0.,-1.,0.));
#1619=DIRECTION('',(0.,0.,1.));
#1620=DIRECTION('',(0.,-1.,0.));
#1621=DIRECTION('',(0.,0.,1.));
#1622=DIRECTION('center_axis',(0.,1.,0.));
#1623=DIRECTION('ref_axis',(0.,0.,1.));
#1624=DIRECTION('',(-1.,0.,0.));
#1625=DIRECTION('',(0.,0.,1.));
#1626=DIRECTION('',(-1.,0.,0.));
#1627=DIRECTION('center_axis',(-1.,0.,0.));
#1628=DIRECTION('ref_axis',(0.,0.,1.));
#1629=DIRECTION('',(0.,-1.,0.));
#1630=DIRECTION('',(0.,0.,1.));
#1631=DIRECTION('',(0.,-1.,0.));
#1632=DIRECTION('center_axis',(0.,-1.,0.));
#1633=DIRECTION('ref_axis',(0.,0.,-1.));
#1634=DIRECTION('',(1.,0.,0.));
#1635=DIRECTION('',(1.,0.,0.));
#1636=DIRECTION('',(0.,0.,1.));
#1637=DIRECTION('',(1.,0.,0.));
#1638=DIRECTION('center_axis',(0.,1.,0.));
#1639=DIRECTION('ref_axis',(0.,0.,1.));
#1640=DIRECTION('',(-1.,0.,0.));
#1641=DIRECTION('',(0.,0.,1.));
#1642=DIRECTION('',(-1.,0.,0.));
#1643=DIRECTION('',(0.,0.,-1.));
#1644=DIRECTION('',(1.,0.,0.));
#1645=DIRECTION('center_axis',(0.707106781186548,0.707106781186548,0.));
#1646=DIRECTION('ref_axis',(-0.707106781186548,0.707106781186548,0.));
#1647=DIRECTION('',(-0.707106781186547,0.707106781186547,0.));
#1648=DIRECTION('',(0.,0.,1.));
#1649=DIRECTION('',(-0.707106781186547,0.707106781186547,0.));
#1650=DIRECTION('center_axis',(1.,0.,0.));
#1651=DIRECTION('ref_axis',(0.,0.,-1.));
#1652=DIRECTION('',(0.,1.,0.));
#1653=DIRECTION('',(0.,0.,1.));
#1654=DIRECTION('',(0.,1.,0.));
#1655=DIRECTION('center_axis',(0.,1.,0.));
#1656=DIRECTION('ref_axis',(0.,0.,1.));
#1657=DIRECTION('',(-1.,0.,0.));
#1658=DIRECTION('',(0.,0.,1.));
#1659=DIRECTION('',(-1.,0.,0.));
#1660=DIRECTION('center_axis',(-1.,0.,0.));
#1661=DIRECTION('ref_axis',(0.,0.,1.));
#1662=DIRECTION('',(0.,-1.,0.));
#1663=DIRECTION('',(0.,0.,1.));
#1664=DIRECTION('',(0.,-1.,0.));
#1665=DIRECTION('center_axis',(-0.707106781186548,0.707106781186548,0.));
#1666=DIRECTION('ref_axis',(-0.707106781186548,-0.707106781186548,0.));
#1667=DIRECTION('',(-0.707106781186547,-0.707106781186547,0.));
#1668=DIRECTION('',(0.,0.,1.));
#1669=DIRECTION('',(-0.707106781186547,-0.707106781186547,0.));
#1670=DIRECTION('center_axis',(0.,1.,0.));
#1671=DIRECTION('ref_axis',(0.,0.,1.));
#1672=DIRECTION('',(-1.,0.,0.));
#1673=DIRECTION('',(-1.,0.,0.));
#1674=DIRECTION('',(0.,0.,1.));
#1675=DIRECTION('',(-1.,0.,0.));
#1676=DIRECTION('center_axis',(0.,-1.,0.));
#1677=DIRECTION('ref_axis',(0.,0.,-1.));
#1678=DIRECTION('',(1.,0.,0.));
#1679=DIRECTION('',(0.,0.,1.));
#1680=DIRECTION('',(1.,0.,0.));
#1681=DIRECTION('',(0.,0.,-1.));
#1682=DIRECTION('',(-1.,0.,0.));
#1683=DIRECTION('center_axis',(0.999999999999972,-2.35372237672442E-7,0.));
#1684=DIRECTION('ref_axis',(2.35372237672442E-7,0.999999999999972,0.));
#1685=DIRECTION('',(2.35372237672442E-7,0.999999999999972,0.));
#1686=DIRECTION('',(0.,0.,1.));
#1687=DIRECTION('',(2.35372237672442E-7,0.999999999999972,0.));
#1688=DIRECTION('center_axis',(0.,1.,0.));
#1689=DIRECTION('ref_axis',(0.,0.,1.));
#1690=DIRECTION('',(-1.,0.,0.));
#1691=DIRECTION('',(0.,0.,1.));
#1692=DIRECTION('',(-1.,0.,0.));
#1693=DIRECTION('center_axis',(1.,0.,0.));
#1694=DIRECTION('ref_axis',(0.,0.,-1.));
#1695=DIRECTION('',(0.,1.,0.));
#1696=DIRECTION('',(0.,0.,1.));
#1697=DIRECTION('',(0.,1.,0.));
#1698=DIRECTION('center_axis',(0.,-1.,0.));
#1699=DIRECTION('ref_axis',(0.,0.,-1.));
#1700=DIRECTION('',(1.,0.,0.));
#1701=DIRECTION('',(0.,0.,1.));
#1702=DIRECTION('',(1.,0.,0.));
#1703=DIRECTION('center_axis',(-0.866025403784439,0.5,0.));
#1704=DIRECTION('ref_axis',(-0.5,-0.866025403784439,0.));
#1705=DIRECTION('',(-0.5,-0.866025403784439,0.));
#1706=DIRECTION('',(0.,0.,1.));
#1707=DIRECTION('',(-0.5,-0.866025403784439,0.));
#1708=DIRECTION('center_axis',(0.,-1.,0.));
#1709=DIRECTION('ref_axis',(0.,0.,-1.));
#1710=DIRECTION('',(1.,0.,0.));
#1711=DIRECTION('',(0.,0.,1.));
#1712=DIRECTION('',(1.,0.,0.));
#1713=DIRECTION('center_axis',(0.866025403784439,0.5,0.));
#1714=DIRECTION('ref_axis',(-0.5,0.866025403784439,0.));
#1715=DIRECTION('',(-0.5,0.866025403784439,0.));
#1716=DIRECTION('',(0.,0.,1.));
#1717=DIRECTION('',(-0.5,0.866025403784439,0.));
#1718=DIRECTION('center_axis',(0.,-1.,0.));
#1719=DIRECTION('ref_axis',(0.,0.,-1.));
#1720=DIRECTION('',(1.,0.,0.));
#1721=DIRECTION('',(1.,0.,0.));
#1722=DIRECTION('center_axis',(0.,0.,-1.));
#1723=DIRECTION('ref_axis',(-1.,0.,0.));
#1724=DIRECTION('',(0.,-1.,0.));
#1725=DIRECTION('',(0.,1.,0.));
#1726=DIRECTION('center_axis',(0.,0.,-1.));
#1727=DIRECTION('ref_axis',(-1.,0.,0.));
#1728=DIRECTION('center_axis',(0.,0.,-1.));
#1729=DIRECTION('ref_axis',(-1.,0.,0.));
#1730=DIRECTION('',(0.,-1.,0.));
#1731=DIRECTION('center_axis',(1.,0.,0.));
#1732=DIRECTION('ref_axis',(0.,0.,-1.));
#1733=DIRECTION('center_axis',(0.,0.,-1.));
#1734=DIRECTION('ref_axis',(-1.,0.,0.));
#1735=DIRECTION('',(0.,1.,0.));
#1736=DIRECTION('center_axis',(1.,0.,0.));
#1737=DIRECTION('ref_axis',(0.,0.,-1.));
#1996=CARTESIAN_POINT('',(0.,0.,0.));
#1997=CARTESIAN_POINT('Origin',(-36.9999998586142,28.9943965601659,-119.188676592855));
#1998=CARTESIAN_POINT('',(-36.9999998586142,52.994396560166,-89.1886765928545));
#1999=CARTESIAN_POINT('',(-36.9999998586142,52.994396560166,40.8113234071455));
#2000=CARTESIAN_POINT('',(-36.9999998586142,52.994396560166,-119.188676592855));
#2001=CARTESIAN_POINT('',(-36.9999998586142,28.9943965601659,-89.1886765928545));
#2002=CARTESIAN_POINT('',(-36.9999998586142,52.994396560166,-89.1886765928545));
#2003=CARTESIAN_POINT('',(-36.9999998586142,28.9943965601659,40.8113234071455));
#2004=CARTESIAN_POINT('',(-36.9999998586142,28.9943965601659,-119.188676592855));
#2005=CARTESIAN_POINT('',(-36.9999998586142,28.9943965601659,40.8113234071455));
#2006=CARTESIAN_POINT('Origin',(37.0000001413876,28.9943965606416,-119.188676592855));
#2007=CARTESIAN_POINT('',(37.0000001413876,28.9943965606416,-89.1886765928545));
#2008=CARTESIAN_POINT('',(37.0000001413876,28.9943965606416,40.8113234071455));
#2009=CARTESIAN_POINT('',(37.0000001413876,28.9943965606416,-119.188676592855));
#2010=CARTESIAN_POINT('',(37.0000001413876,52.9943965606364,-89.1886765928545));
#2011=CARTESIAN_POINT('',(37.0000001413876,52.9943965606364,-89.1886765928545));
#2012=CARTESIAN_POINT('',(37.0000001413876,52.9943965606364,40.8113234071455));
#2013=CARTESIAN_POINT('',(37.0000001413876,52.9943965606364,-119.188676592855));
#2014=CARTESIAN_POINT('',(37.0000001413876,28.9943965606416,40.8113234071455));
#2015=CARTESIAN_POINT('Origin',(-49.9999998586142,-15.0056034398341,-119.188676592855));
#2016=CARTESIAN_POINT('',(-49.9999998586142,8.99439656016592,40.8113234071455));
#2017=CARTESIAN_POINT('',(-49.9999998586142,-15.0056034398341,40.8113234071455));
#2018=CARTESIAN_POINT('',(-49.9999998586142,-15.0056034398341,40.8113234071455));
#2019=CARTESIAN_POINT('',(-49.9999998586142,8.99439656016592,-119.188676592855));
#2020=CARTESIAN_POINT('',(-49.9999998586142,8.99439656016592,-119.188676592855));
#2021=CARTESIAN_POINT('',(-49.9999998586142,-15.0056034398341,-119.188676592855));
#2022=CARTESIAN_POINT('',(-49.9999998586142,-15.0056034398341,-119.188676592855));
#2023=CARTESIAN_POINT('',(-49.9999998586142,-15.0056034398341,-119.188676592855));
#2024=CARTESIAN_POINT('Origin',(-49.9999998586142,8.99439656016592,-119.188676592855));
#2025=CARTESIAN_POINT('',(-25.9999998586142,8.99439656016592,40.8113234071455));
#2026=CARTESIAN_POINT('',(-49.9999998586142,8.99439656016592,40.8113234071455));
#2027=CARTESIAN_POINT('',(-25.9999998586142,8.99439656016592,-119.188676592855));
#2028=CARTESIAN_POINT('',(-25.9999998586142,8.99439656016592,-119.188676592855));
#2029=CARTESIAN_POINT('',(-49.9999998586142,8.99439656016592,-119.188676592855));
#2030=CARTESIAN_POINT('Origin',(-25.9999998586142,8.99439656016592,-119.188676592855));
#2031=CARTESIAN_POINT('',(-25.9999998586142,28.9943965601659,40.8113234071455));
#2032=CARTESIAN_POINT('',(-25.9999998586142,8.99439656016592,40.8113234071455));
#2033=CARTESIAN_POINT('',(-25.9999998586142,28.9943965601659,-119.188676592855));
#2034=CARTESIAN_POINT('',(-25.9999998586142,28.9943965601659,-119.188676592855));
#2035=CARTESIAN_POINT('',(-25.9999998586142,8.99439656016592,-119.188676592855));
#2036=CARTESIAN_POINT('Origin',(-25.9999998586142,28.9943965601659,-119.188676592855));
#2037=CARTESIAN_POINT('',(-25.9999998586142,28.9943965601659,40.8113234071455));
#2038=CARTESIAN_POINT('',(-48.9999998586142,28.9943965601659,-89.1886765928545));
#2039=CARTESIAN_POINT('',(-48.9999998586142,28.9943965601659,-89.1886765928545));
#2040=CARTESIAN_POINT('',(-48.9999998586142,28.9943965601659,-119.188676592855));
#2041=CARTESIAN_POINT('',(-48.9999998586142,28.9943965601659,-89.1886765928545));
#2042=CARTESIAN_POINT('',(-25.9999998586142,28.9943965601659,-119.188676592855));
#2043=CARTESIAN_POINT('Origin',(-36.9999998586142,52.994396560166,-119.188676592855));
#2044=CARTESIAN_POINT('',(-24.9999998586142,52.994396560166,40.8113234071455));
#2045=CARTESIAN_POINT('',(-36.9999998586142,52.994396560166,40.8113234071455));
#2046=CARTESIAN_POINT('',(-24.9999998586142,52.994396560166,-119.188676592855));
#2047=CARTESIAN_POINT('',(-24.9999998586142,52.994396560166,-119.188676592855));
#2048=CARTESIAN_POINT('',(-48.9999998586142,52.994396560166,-119.188676592855));
#2049=CARTESIAN_POINT('',(-36.9999998586142,52.994396560166,-119.188676592855));
#2050=CARTESIAN_POINT('',(-48.9999998586142,52.994396560166,-89.1886765928545));
#2051=CARTESIAN_POINT('',(-48.9999998586142,52.994396560166,-119.188676592855));
#2052=CARTESIAN_POINT('',(-48.9999998586142,52.994396560166,-89.1886765928545));
#2053=CARTESIAN_POINT('Origin',(-24.9999998586142,52.994396560166,-119.188676592855));
#2054=CARTESIAN_POINT('',(-2.99999985861422,30.994396560166,40.8113234071455));
#2055=CARTESIAN_POINT('',(-24.9999998586142,52.994396560166,40.8113234071455));
#2056=CARTESIAN_POINT('',(-2.99999985861422,30.994396560166,-119.188676592855));
#2057=CARTESIAN_POINT('',(-2.99999985861422,30.994396560166,-119.188676592855));
#2058=CARTESIAN_POINT('',(-24.9999998586142,52.994396560166,-119.188676592855));
#2059=CARTESIAN_POINT('Origin',(-2.99999985861422,30.994396560166,-119.188676592855));
#2060=CARTESIAN_POINT('',(-2.99999985861422,26.9943965601665,40.8113234071455));
#2061=CARTESIAN_POINT('',(-2.99999985861422,30.994396560166,40.8113234071455));
#2062=CARTESIAN_POINT('',(-2.99999985861422,26.9943965601665,-119.188676592855));
#2063=CARTESIAN_POINT('',(-2.99999985861422,26.9943965601665,-119.188676592855));
#2064=CARTESIAN_POINT('',(-2.99999985861422,30.994396560166,-119.188676592855));
#2065=CARTESIAN_POINT('Origin',(-2.99999985861422,26.9943965601665,-119.188676592855));
#2066=CARTESIAN_POINT('',(3.00000014138191,26.9943965601665,40.8113234071455));
#2067=CARTESIAN_POINT('',(-2.99999985861422,26.9943965601665,40.8113234071455));
#2068=CARTESIAN_POINT('',(3.00000014138191,26.9943965601665,-119.188676592855));
#2069=CARTESIAN_POINT('',(3.00000014138191,26.9943965601665,-119.188676592855));
#2070=CARTESIAN_POINT('',(-2.99999985861422,26.9943965601665,-119.188676592855));
#2071=CARTESIAN_POINT('Origin',(3.00000014138191,30.9943965606328,-119.188676592855));
#2072=CARTESIAN_POINT('',(3.00000014138191,30.9943965606328,40.8113234071455));
#2073=CARTESIAN_POINT('',(3.00000014138191,30.9943965606328,40.8113234071455));
#2074=CARTESIAN_POINT('',(3.00000014138191,30.9943965606328,-119.188676592855));
#2075=CARTESIAN_POINT('',(3.00000014138191,30.9943965606328,-119.188676592855));
#2076=CARTESIAN_POINT('',(3.00000014138191,30.9943965606328,-119.188676592855));
#2077=CARTESIAN_POINT('Origin',(25.0000001413855,52.9943965606364,-119.188676592855));
#2078=CARTESIAN_POINT('',(25.0000001413855,52.9943965606364,40.8113234071455));
#2079=CARTESIAN_POINT('',(25.0000001413855,52.9943965606364,40.8113234071455));
#2080=CARTESIAN_POINT('',(25.0000001413855,52.9943965606364,-119.188676592855));
#2081=CARTESIAN_POINT('',(25.0000001413855,52.9943965606364,-119.188676592855));
#2082=CARTESIAN_POINT('',(25.0000001413855,52.9943965606364,-119.188676592855));
#2083=CARTESIAN_POINT('Origin',(37.0000001413876,52.9943965606364,-119.188676592855));
#2084=CARTESIAN_POINT('',(37.0000001413876,52.9943965606364,40.8113234071455));
#2085=CARTESIAN_POINT('',(49.0000001413876,52.9943965606364,-89.1886765928545));
#2086=CARTESIAN_POINT('',(49.0000001413876,52.9943965606364,-89.1886765928545));
#2087=CARTESIAN_POINT('',(49.0000001413876,52.9943965606364,-119.188676592855));
#2088=CARTESIAN_POINT('',(49.0000001413876,52.9943965606364,-119.188676592855));
#2089=CARTESIAN_POINT('',(37.0000001413876,52.9943965606364,-119.188676592855));
#2090=CARTESIAN_POINT('Origin',(26.0000001413871,28.9943965606416,-119.188676592855));
#2091=CARTESIAN_POINT('',(26.0000001413871,28.9943965606416,40.8113234071455));
#2092=CARTESIAN_POINT('',(26.0000001413871,28.9943965606416,40.8113234071455));
#2093=CARTESIAN_POINT('',(26.0000001413871,28.9943965606416,-119.188676592855));
#2094=CARTESIAN_POINT('',(26.0000001413871,28.9943965606416,-119.188676592855));
#2095=CARTESIAN_POINT('',(49.0000001413876,28.9943965606416,-119.188676592855));
#2096=CARTESIAN_POINT('',(26.0000001413871,28.9943965606416,-119.188676592855));
#2097=CARTESIAN_POINT('',(49.0000001413876,28.9943965606416,-89.1886765928545));
#2098=CARTESIAN_POINT('',(49.0000001413876,28.9943965606416,-89.1886765928545));
#2099=CARTESIAN_POINT('',(49.0000001413876,28.9943965606416,-89.1886765928545));
#2100=CARTESIAN_POINT('Origin',(25.9999954339423,8.99439656064154,-119.188676592855));
#2101=CARTESIAN_POINT('',(25.9999954339423,8.99439656064154,40.8113234071455));
#2102=CARTESIAN_POINT('',(25.9999954339423,8.99439656064154,40.8113234071455));
#2103=CARTESIAN_POINT('',(25.9999954339423,8.99439656064154,-119.188676592855));
#2104=CARTESIAN_POINT('',(25.9999954339423,8.99439656064154,-119.188676592855));
#2105=CARTESIAN_POINT('',(25.9999954339423,8.99439656064154,-119.188676592855));
#2106=CARTESIAN_POINT('Origin',(50.0000001413858,8.99439656064154,-119.188676592855));
#2107=CARTESIAN_POINT('',(50.0000001413858,8.99439656064154,40.8113234071455));
#2108=CARTESIAN_POINT('',(50.0000001413858,8.99439656064154,40.8113234071455));
#2109=CARTESIAN_POINT('',(50.0000001413858,8.99439656064154,-119.188676592855));
#2110=CARTESIAN_POINT('',(50.0000001413858,8.99439656064154,-119.188676592855));
#2111=CARTESIAN_POINT('',(50.0000001413858,8.99439656064154,-119.188676592855));
#2112=CARTESIAN_POINT('Origin',(50.0000001413858,-15.0056034398341,-119.188676592855));
#2113=CARTESIAN_POINT('',(50.0000001413858,-15.0056034398341,40.8113234071455));
#2114=CARTESIAN_POINT('',(50.0000001413858,-15.0056034398341,40.8113234071455));
#2115=CARTESIAN_POINT('',(50.0000001413858,-15.0056034398341,-119.188676592855));
#2116=CARTESIAN_POINT('',(50.0000001413858,-15.0056034398341,-119.188676592855));
#2117=CARTESIAN_POINT('',(50.0000001413858,-15.0056034398341,-119.188676592855));
#2118=CARTESIAN_POINT('Origin',(50.0000001413858,-15.0056034398341,-119.188676592855));
#2119=CARTESIAN_POINT('',(15.0000001413858,-15.0056034398341,40.8113234071455));
#2120=CARTESIAN_POINT('',(50.0000001413858,-15.0056034398341,40.8113234071455));
#2121=CARTESIAN_POINT('',(15.0000001413858,-15.0056034398341,-119.188676592855));
#2122=CARTESIAN_POINT('',(15.0000001413858,-15.0056034398341,-119.188676592855));
#2123=CARTESIAN_POINT('',(50.0000001413858,-15.0056034398341,-119.188676592855));
#2124=CARTESIAN_POINT('Origin',(15.0000001413858,-15.0056034398341,-119.188676592855));
#2125=CARTESIAN_POINT('',(20.773502833282,-5.00560343983409,40.8113234071455));
#2126=CARTESIAN_POINT('',(15.0000001413858,-15.0056034398341,40.8113234071455));
#2127=CARTESIAN_POINT('',(20.773502833282,-5.00560343983409,-119.188676592855));
#2128=CARTESIAN_POINT('',(20.773502833282,-5.00560343983409,-119.188676592855));
#2129=CARTESIAN_POINT('',(15.0000001413858,-15.0056034398341,-119.188676592855));
#2130=CARTESIAN_POINT('Origin',(15.0000001413858,-5.00560343983409,-119.188676592855));
#2131=CARTESIAN_POINT('',(-20.7735025505105,-5.00560343983409,40.8113234071455));
#2132=CARTESIAN_POINT('',(15.0000001413858,-5.00560343983409,40.8113234071455));
#2133=CARTESIAN_POINT('',(-20.7735025505105,-5.00560343983409,-119.188676592855));
#2134=CARTESIAN_POINT('',(-20.7735025505105,-5.00560343983409,-119.188676592855));
#2135=CARTESIAN_POINT('',(-14.9999998586142,-5.00560343983409,-119.188676592855));
#2136=CARTESIAN_POINT('Origin',(-14.9999998586142,-15.0056034398341,-119.188676592855));
#2137=CARTESIAN_POINT('',(-14.9999998586142,-15.0056034398341,40.8113234071455));
#2138=CARTESIAN_POINT('',(-14.9999998586142,-15.0056034398341,40.8113234071455));
#2139=CARTESIAN_POINT('',(-14.9999998586142,-15.0056034398341,-119.188676592855));
#2140=CARTESIAN_POINT('',(-14.9999998586142,-15.0056034398341,-119.188676592855));
#2141=CARTESIAN_POINT('',(-14.9999998586142,-15.0056034398341,-119.188676592855));
#2142=CARTESIAN_POINT('Origin',(-49.9999998586142,-15.0056034398341,-119.188676592855));
#2143=CARTESIAN_POINT('',(-49.9999998586142,-15.0056034398341,40.8113234071455));
#2144=CARTESIAN_POINT('',(-49.9999998586142,-15.0056034398341,-119.188676592855));
#2145=CARTESIAN_POINT('Origin',(1.41385779953466E-7,-15.0056034398341,-119.188676592855));
#2146=CARTESIAN_POINT('',(-48.9999998586142,28.9943965601659,-119.188676592855));
#2147=CARTESIAN_POINT('',(49.0000001413876,28.9943965606416,-119.188676592855));
#2148=CARTESIAN_POINT('Origin',(1.41385779953466E-7,-15.0056034398341,40.8113234071455));
#2149=CARTESIAN_POINT('Origin',(49.0000001413876,52.9943965606364,-89.1886765928545));
#2150=CARTESIAN_POINT('',(49.0000001413876,52.9943965606364,-89.1886765928545));
#2151=CARTESIAN_POINT('Origin',(49.0000001413876,-15.0056034398341,40.8113234071455));
#2152=CARTESIAN_POINT('Origin',(-48.9999998586142,52.994396560166,-89.1886765928545));
#2153=CARTESIAN_POINT('',(-48.9999998586142,52.994396560166,-89.1886765928545));
#2154=CARTESIAN_POINT('Origin',(-48.9999998586142,-15.0056034398341,40.8113234071455));
#2467=UNCERTAINTY_MEASURE_WITH_UNIT(LENGTH_MEASURE(0.01),#2478,
'DISTANCE_ACCURACY_VALUE',
'Maximum model space distance between geometric entities at asserted c
onnectivities');
#2471=UNCERTAINTY_MEASURE_WITH_UNIT(LENGTH_MEASURE(0.01),#2478,
'DISTANCE_ACCURACY_VALUE',
'Maximum model space distance between geometric entities at asserted c
onnectivities');
#2473=(
GEOMETRIC_REPRESENTATION_CONTEXT(3)
GLOBAL_UNCERTAINTY_ASSIGNED_CONTEXT((#2467))
GLOBAL_UNIT_ASSIGNED_CONTEXT((#2478,#2480,#2481))
REPRESENTATION_CONTEXT('','3D')
);
#2477=(
GEOMETRIC_REPRESENTATION_CONTEXT(3)
GLOBAL_UNCERTAINTY_ASSIGNED_CONTEXT((#2471))
GLOBAL_UNIT_ASSIGNED_CONTEXT((#2478,#2480,#2481))
REPRESENTATION_CONTEXT('','3D')
);
#2478=(
LENGTH_UNIT()
NAMED_UNIT(*)
SI_UNIT(.MILLI.,.METRE.)
);
#2480=(
NAMED_UNIT(*)
PLANE_ANGLE_UNIT()
SI_UNIT($,.RADIAN.)
);
#2481=(
NAMED_UNIT(*)
SI_UNIT($,.STERADIAN.)
SOLID_ANGLE_UNIT()
);
#2483=SHAPE_DEFINITION_REPRESENTATION(#2488,#2497);
#2488=PRODUCT_DEFINITION_SHAPE('',$,#2503);
#2497=SHAPE_REPRESENTATION('',(#1477),#2473);
#2501=PRODUCT_DEFINITION_CONTEXT('part definition',#2518,'design');
#2503=PRODUCT_DEFINITION('V-Block','V-Block',#2508,#2501);
#2508=PRODUCT_DEFINITION_FORMATION('',$,#2521);
#2518=APPLICATION_CONTEXT(
'Core Data for Automotive Mechanical Design Process');
#2519=PRODUCT_CONTEXT('part definition',#2518,'mechanical');
#2521=PRODUCT('V-Block','V-Block',$,(#2519));
#2526=PRESENTATION_STYLE_ASSIGNMENT((#2531));
#2531=SURFACE_STYLE_USAGE(.BOTH.,#2536);
#2536=SURFACE_SIDE_STYLE('',(#2541));
#2541=SURFACE_STYLE_FILL_AREA(#2546);
#2546=FILL_AREA_STYLE('Opaque(97,158,199)',(#2551));
#2551=FILL_AREA_STYLE_COLOUR('Opaque(97,158,199)',#2556);
#2556=COLOUR_RGB('Opaque(97,158,199)',0.380392156862745,0.619607843137255,
0.780392156862745);
ENDSEC;
END-ISO-10303-21;
